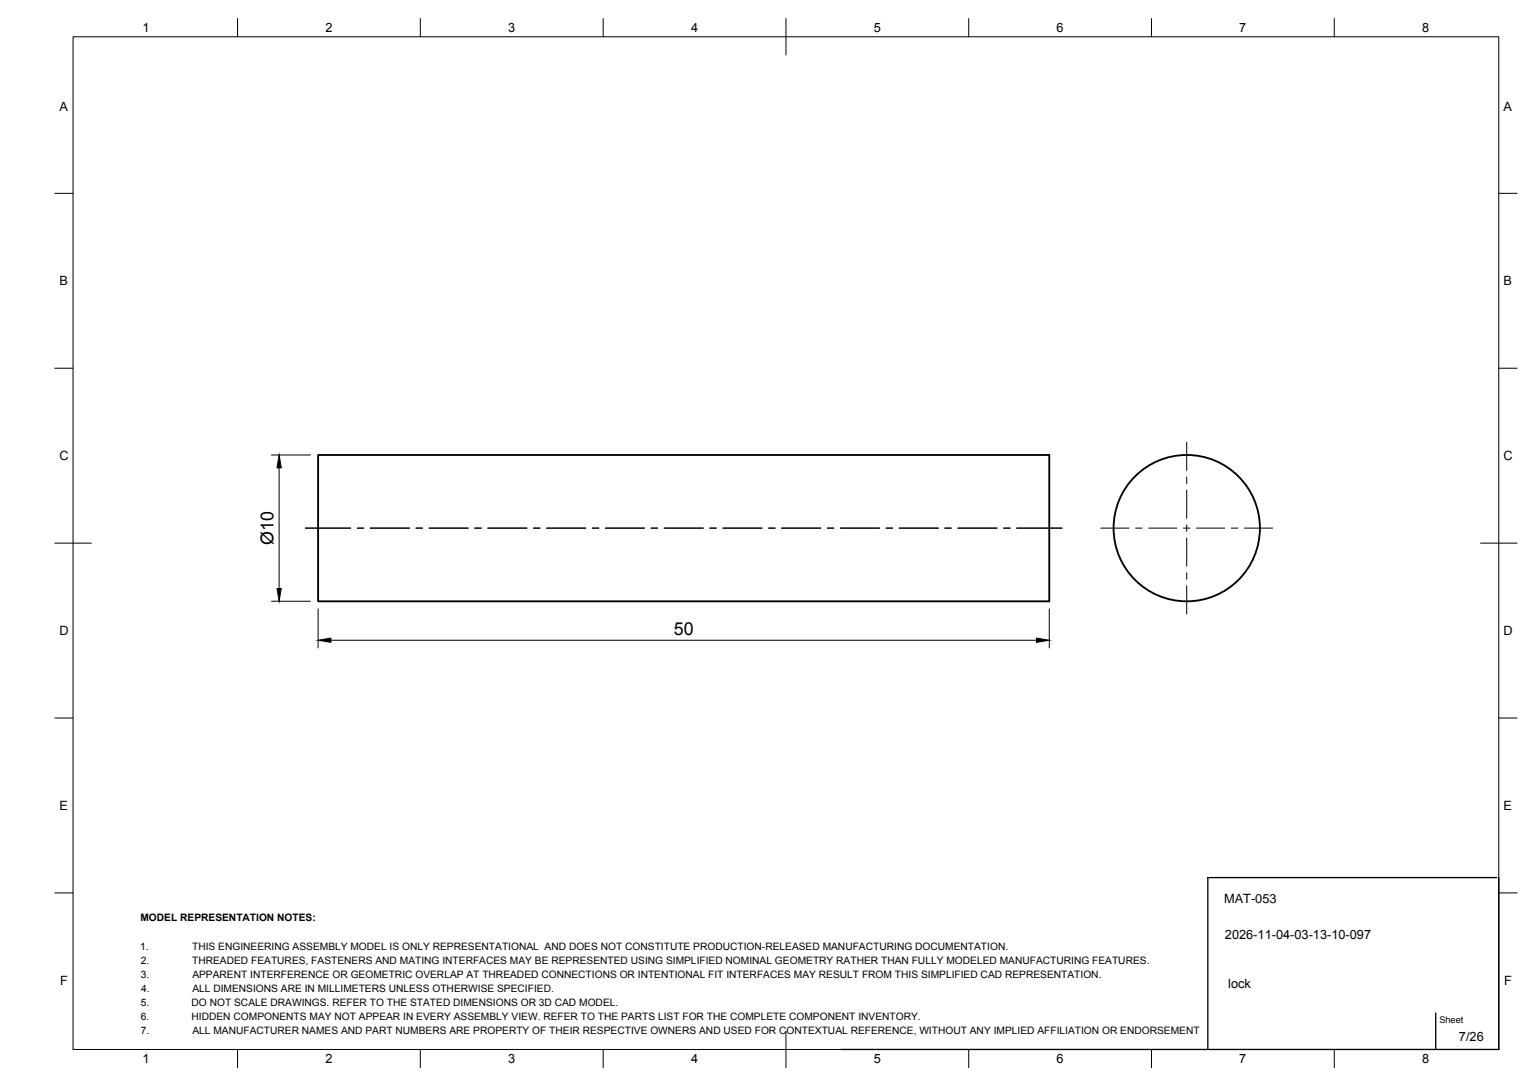
ISO-10303-21;
HEADER;
FILE_DESCRIPTION (('STEP AP214'),
    '1' );
FILE_NAME ('lock.step',
    '2026-10-10T03:43:58',
    ( '' ),
    ( '' ),
    'SwSTEP 2.0',
    'SolidWorks 2026',
    '' );
FILE_SCHEMA (( 'AUTOMOTIVE_DESIGN' ));
ENDSEC;

DATA;
#244=PRESENTATION_STYLE_ASSIGNMENT (( #27321 ) ) ;
#620=CARTESIAN_POINT ( 'NONE',  ( 0.000000000000000000, 0.000000000000000000, 0.000000000000000000 ) ) ;
#994=LINE ( 'NONE', #43880, #49914 ) ;
#1824=ORIENTED_EDGE ( 'NONE', *, *, #5705, .T. ) ;
#1832=ADVANCED_FACE ( 'NONE', ( #65660 ), #28357, .T. ) ;
#1876=EDGE_CURVE ( 'NONE', #59383, #13453, #2673, .T. ) ;
#1922=EDGE_CURVE ( 'NONE', #13453, #38828, #44149, .T. ) ;
#2673=LINE ( 'NONE', #25526, #4850 ) ;
#4574=EDGE_CURVE ( 'NONE', #38828, #13453, #27371, .T. ) ;
#4850=VECTOR ( 'NONE', #46965, 1000.000000000000000 ) ;
#5705=EDGE_CURVE ( 'NONE', #59383, #9126, #28554, .T. ) ;
#6925=SURFACE_STYLE_FILL_AREA ( #22753 ) ;
#8047=DIRECTION ( 'NONE',  ( 0.000000000000000000, 1.000000000000000000, 0.000000000000000000 ) ) ;
#8319=DIRECTION ( 'NONE',  ( 1.000000000000000000, 0.000000000000000000, 0.000000000000000000 ) ) ;
#8668=( NAMED_UNIT ( * ) PLANE_ANGLE_UNIT ( ) SI_UNIT ( $, .RADIAN. ) );
#9126=VERTEX_POINT ( 'NONE', #28099 ) ;
#10441=COLOUR_RGB ( '',0.7921568627450980005, 0.8196078431372548767, 0.9333333333333333481 ) ;
#10468=AXIS2_PLACEMENT_3D ( 'NONE', #39958, #11829, #34698 ) ;
#10569=ADVANCED_BREP_SHAPE_REPRESENTATION ( '', ( #41060, #66832 ), #12941 ) ;
#11313=PRODUCT_DEFINITION_CONTEXT ( 'detailed design', #58366, 'design' ) ;
#11829=DIRECTION ( 'NONE',  ( 0.000000000000000000, 1.000000000000000000, 0.000000000000000000 ) ) ;
#12109=ORIENTED_EDGE ( 'NONE', *, *, #39188, .T. ) ;
#12753=CARTESIAN_POINT ( 'NONE',  ( 0.000000000000000000, 0.000000000000000000, -5.000000000000000000 ) ) ;
#12941=( GEOMETRIC_REPRESENTATION_CONTEXT ( 3 ) GLOBAL_UNCERTAINTY_ASSIGNED_CONTEXT ( ( #50779 ) ) GLOBAL_UNIT_ASSIGNED_CONTEXT ( ( #35744, #8668, #15315 ) ) REPRESENTATION_CONTEXT ( 'NONE', 'WORKASPACE' ) );
#13336=PLANE ( 'NONE',  #42927 ) ;
#13453=VERTEX_POINT ( 'NONE', #57768 ) ;
#14709=DIRECTION ( 'NONE',  ( -0.000000000000000000, -1.000000000000000000, -0.000000000000000000 ) ) ;
#14930=AXIS2_PLACEMENT_3D ( 'NONE', #47917, #32103, #25462 ) ;
#14987=AXIS2_PLACEMENT_3D ( 'NONE', #620, #60405, #60043 ) ;
#15315=( NAMED_UNIT ( * ) SI_UNIT ( $, .STERADIAN. ) SOLID_ANGLE_UNIT ( ) );
#15585=CYLINDRICAL_SURFACE ( 'NONE', #14930, 5.000000000000000000 ) ;
#15765=ORIENTED_EDGE ( 'NONE', *, *, #39188, .F. ) ;
#16024=DIRECTION ( 'NONE',  ( 0.000000000000000000, 0.000000000000000000, 1.000000000000000000 ) ) ;
#16405=DIRECTION ( 'NONE',  ( 0.000000000000000000, 0.000000000000000000, 1.000000000000000000 ) ) ;
#16674=EDGE_LOOP ( 'NONE', ( #43350, #15765, #37484, #21366 ) ) ;
#16771=( NAMED_UNIT ( * ) SI_UNIT ( $, .STERADIAN. ) SOLID_ANGLE_UNIT ( ) );
#17832=( LENGTH_UNIT ( ) NAMED_UNIT ( * ) SI_UNIT ( .MILLI., .METRE. ) );
#17920=APPLICATION_CONTEXT ( 'automotive_design' ) ;
#19523=SHAPE_REPRESENTATION ( 'lock', ( #66832 ), #12941 ) ;
#20241=SHAPE_REPRESENTATION_RELATIONSHIP ( 'NONE' , 'NONE' ,  #19523, #10569 ) ;
#21366=ORIENTED_EDGE ( 'NONE', *, *, #4574, .T. ) ;
#21561=CLOSED_SHELL ( 'NONE', ( #53740, #29963, #1832, #53099 ) ) ;
#21603=DIRECTION ( 'NONE',  ( 0.000000000000000000, 0.000000000000000000, 1.000000000000000000 ) ) ;
#21915=ORIENTED_EDGE ( 'NONE', *, *, #1922, .T. ) ;
#22753=FILL_AREA_STYLE ('',( #64976 ) ) ;
#23878=AXIS2_PLACEMENT_3D ( 'NONE', #64598, #27996, #16405 ) ;
#24926=FACE_OUTER_BOUND ( 'NONE', #65253, .T. ) ;
#25081=( GEOMETRIC_REPRESENTATION_CONTEXT ( 3 ) GLOBAL_UNCERTAINTY_ASSIGNED_CONTEXT ( ( #61342 ) ) GLOBAL_UNIT_ASSIGNED_CONTEXT ( ( #17832, #44191, #16771 ) ) REPRESENTATION_CONTEXT ( 'NONE', 'WORKASPACE' ) );
#25278=DIRECTION ( 'NONE',  ( 0.000000000000000000, -0.000000000000000000, 1.000000000000000000 ) ) ;
#25462=DIRECTION ( 'NONE',  ( 0.000000000000000000, 0.000000000000000000, -1.000000000000000000 ) ) ;
#25526=CARTESIAN_POINT ( 'NONE',  ( 6.123233995736766282E-16, 50.00000000000000000, 5.000000000000000000 ) ) ;
#27321=SURFACE_STYLE_USAGE ( .BOTH. , #48412 ) ;
#27371=CIRCLE ( 'NONE', #14987, 5.000000000000000000 ) ;
#27996=DIRECTION ( 'NONE',  ( 0.000000000000000000, 1.000000000000000000, 0.000000000000000000 ) ) ;
#28062=DIRECTION ( 'NONE',  ( -0.000000000000000000, -1.000000000000000000, -0.000000000000000000 ) ) ;
#28099=CARTESIAN_POINT ( 'NONE',  ( 0.000000000000000000, 50.00000000000000000, -5.000000000000000000 ) ) ;
#28232=PRODUCT ( 'lock', 'lock', '', ( #69469 ) ) ;
#28357=PLANE ( 'NONE',  #10468 ) ;
#28554=CIRCLE ( 'NONE', #67879, 5.000000000000000000 ) ;
#28900=PRODUCT_DEFINITION ( 'UNKNOWN', '', #62490, #11313 ) ;
#29094=ORIENTED_EDGE ( 'NONE', *, *, #42402, .F. ) ;
#29963=ADVANCED_FACE ( 'NONE', ( #64276 ), #30546, .T. ) ;
#29988=AXIS2_PLACEMENT_3D ( 'NONE', #51997, #14709, #68851 ) ;
#30546=CYLINDRICAL_SURFACE ( 'NONE', #29988, 5.000000000000000000 ) ;
#31523=DIRECTION ( 'NONE',  ( 0.000000000000000000, 1.000000000000000000, 0.000000000000000000 ) ) ;
#31815=AXIS2_PLACEMENT_3D ( 'NONE', #69447, #69093, #21603 ) ;
#32103=DIRECTION ( 'NONE',  ( -0.000000000000000000, -1.000000000000000000, -0.000000000000000000 ) ) ;
#34698=DIRECTION ( 'NONE',  ( 0.000000000000000000, -0.000000000000000000, 1.000000000000000000 ) ) ;
#35744=( LENGTH_UNIT ( ) NAMED_UNIT ( * ) SI_UNIT ( .MILLI., .METRE. ) );
#37484=ORIENTED_EDGE ( 'NONE', *, *, #42402, .T. ) ;
#38794=ORIENTED_EDGE ( 'NONE', *, *, #5705, .F. ) ;
#38828=VERTEX_POINT ( 'NONE', #12753 ) ;
#39188=EDGE_CURVE ( 'NONE', #9126, #59383, #54159, .T. ) ;
#39958=CARTESIAN_POINT ( 'NONE',  ( 0.000000000000000000, 50.00000000000000000, 0.000000000000000000 ) ) ;
#40446=ORIENTED_EDGE ( 'NONE', *, *, #4574, .F. ) ;
#41060=MANIFOLD_SOLID_BREP ( 'Boss-Extrude1', #21561 ) ;
#42402=EDGE_CURVE ( 'NONE', #9126, #38828, #994, .T. ) ;
#42927=AXIS2_PLACEMENT_3D ( 'NONE', #50962, #8047, #25278 ) ;
#43350=ORIENTED_EDGE ( 'NONE', *, *, #1876, .F. ) ;
#43427=EDGE_LOOP ( 'NONE', ( #38794, #66431, #21915, #29094 ) ) ;
#43880=CARTESIAN_POINT ( 'NONE',  ( 0.000000000000000000, 50.00000000000000000, -5.000000000000000000 ) ) ;
#44149=CIRCLE ( 'NONE', #31815, 5.000000000000000000 ) ;
#44191=( NAMED_UNIT ( * ) PLANE_ANGLE_UNIT ( ) SI_UNIT ( $, .RADIAN. ) );
#44558=DIRECTION ( 'NONE',  ( 0.000000000000000000, 0.000000000000000000, 1.000000000000000000 ) ) ;
#46399=STYLED_ITEM ( 'NONE', ( #244 ), #41060 ) ;
#46965=DIRECTION ( 'NONE',  ( -0.000000000000000000, -1.000000000000000000, -0.000000000000000000 ) ) ;
#47568=FACE_OUTER_BOUND ( 'NONE', #43427, .T. ) ;
#47917=CARTESIAN_POINT ( 'NONE',  ( 0.000000000000000000, 50.00000000000000000, 0.000000000000000000 ) ) ;
#48412=SURFACE_SIDE_STYLE ('',( #6925 ) ) ;
#49750=MECHANICAL_DESIGN_GEOMETRIC_PRESENTATION_REPRESENTATION('',(#46399),#25081);
#49914=VECTOR ( 'NONE', #28062, 1000.000000000000000 ) ;
#50530=CARTESIAN_POINT ( 'NONE',  ( 0.000000000000000000, 0.000000000000000000, 0.000000000000000000 ) ) ;
#50779=UNCERTAINTY_MEASURE_WITH_UNIT (LENGTH_MEASURE( 1.000000000000000082E-05 ), #35744, 'distance_accuracy_value', 'NONE');
#50962=CARTESIAN_POINT ( 'NONE',  ( 0.000000000000000000, 0.000000000000000000, 0.000000000000000000 ) ) ;
#51997=CARTESIAN_POINT ( 'NONE',  ( 0.000000000000000000, 50.00000000000000000, 0.000000000000000000 ) ) ;
#53099=ADVANCED_FACE ( 'NONE', ( #24926 ), #13336, .F. ) ;
#53297=CARTESIAN_POINT ( 'NONE',  ( 0.000000000000000000, 50.00000000000000000, 0.000000000000000000 ) ) ;
#53740=ADVANCED_FACE ( 'NONE', ( #47568 ), #15585, .T. ) ;
#54159=CIRCLE ( 'NONE', #23878, 5.000000000000000000 ) ;
#54614=PRODUCT_DEFINITION_SHAPE ( 'NONE', 'NONE',  #28900 ) ;
#55802=CARTESIAN_POINT ( 'NONE',  ( 6.123233995736766282E-16, 50.00000000000000000, 5.000000000000000000 ) ) ;
#57768=CARTESIAN_POINT ( 'NONE',  ( 6.123233995736766282E-16, 0.000000000000000000, 5.000000000000000000 ) ) ;
#58366=APPLICATION_CONTEXT ( 'automotive_design' ) ;
#58561=SHAPE_DEFINITION_REPRESENTATION ( #54614, #19523 ) ;
#59383=VERTEX_POINT ( 'NONE', #55802 ) ;
#60043=DIRECTION ( 'NONE',  ( 0.000000000000000000, 0.000000000000000000, 1.000000000000000000 ) ) ;
#60405=DIRECTION ( 'NONE',  ( 0.000000000000000000, 1.000000000000000000, 0.000000000000000000 ) ) ;
#61342=UNCERTAINTY_MEASURE_WITH_UNIT (LENGTH_MEASURE( 1.000000000000000082E-05 ), #17832, 'distance_accuracy_value', 'NONE');
#62490=PRODUCT_DEFINITION_FORMATION_WITH_SPECIFIED_SOURCE ( 'ANY', '', #28232, .NOT_KNOWN. ) ;
#64276=FACE_OUTER_BOUND ( 'NONE', #16674, .T. ) ;
#64598=CARTESIAN_POINT ( 'NONE',  ( 0.000000000000000000, 50.00000000000000000, 0.000000000000000000 ) ) ;
#64976=FILL_AREA_STYLE_COLOUR ( '', #10441 ) ;
#65253=EDGE_LOOP ( 'NONE', ( #40446, #67515 ) ) ;
#65614=EDGE_LOOP ( 'NONE', ( #12109, #1824 ) ) ;
#65660=FACE_OUTER_BOUND ( 'NONE', #65614, .T. ) ;
#66431=ORIENTED_EDGE ( 'NONE', *, *, #1876, .T. ) ;
#66832=AXIS2_PLACEMENT_3D ( 'NONE', #50530, #44558, #8319 ) ;
#67515=ORIENTED_EDGE ( 'NONE', *, *, #1922, .F. ) ;
#67879=AXIS2_PLACEMENT_3D ( 'NONE', #53297, #31523, #16024 ) ;
#68851=DIRECTION ( 'NONE',  ( 0.000000000000000000, 0.000000000000000000, -1.000000000000000000 ) ) ;
#69093=DIRECTION ( 'NONE',  ( 0.000000000000000000, 1.000000000000000000, 0.000000000000000000 ) ) ;
#69447=CARTESIAN_POINT ( 'NONE',  ( 0.000000000000000000, 0.000000000000000000, 0.000000000000000000 ) ) ;
#69469=PRODUCT_CONTEXT ( 'NONE', #17920, 'mechanical' ) ;
ENDSEC;
END-ISO-10303-21;
